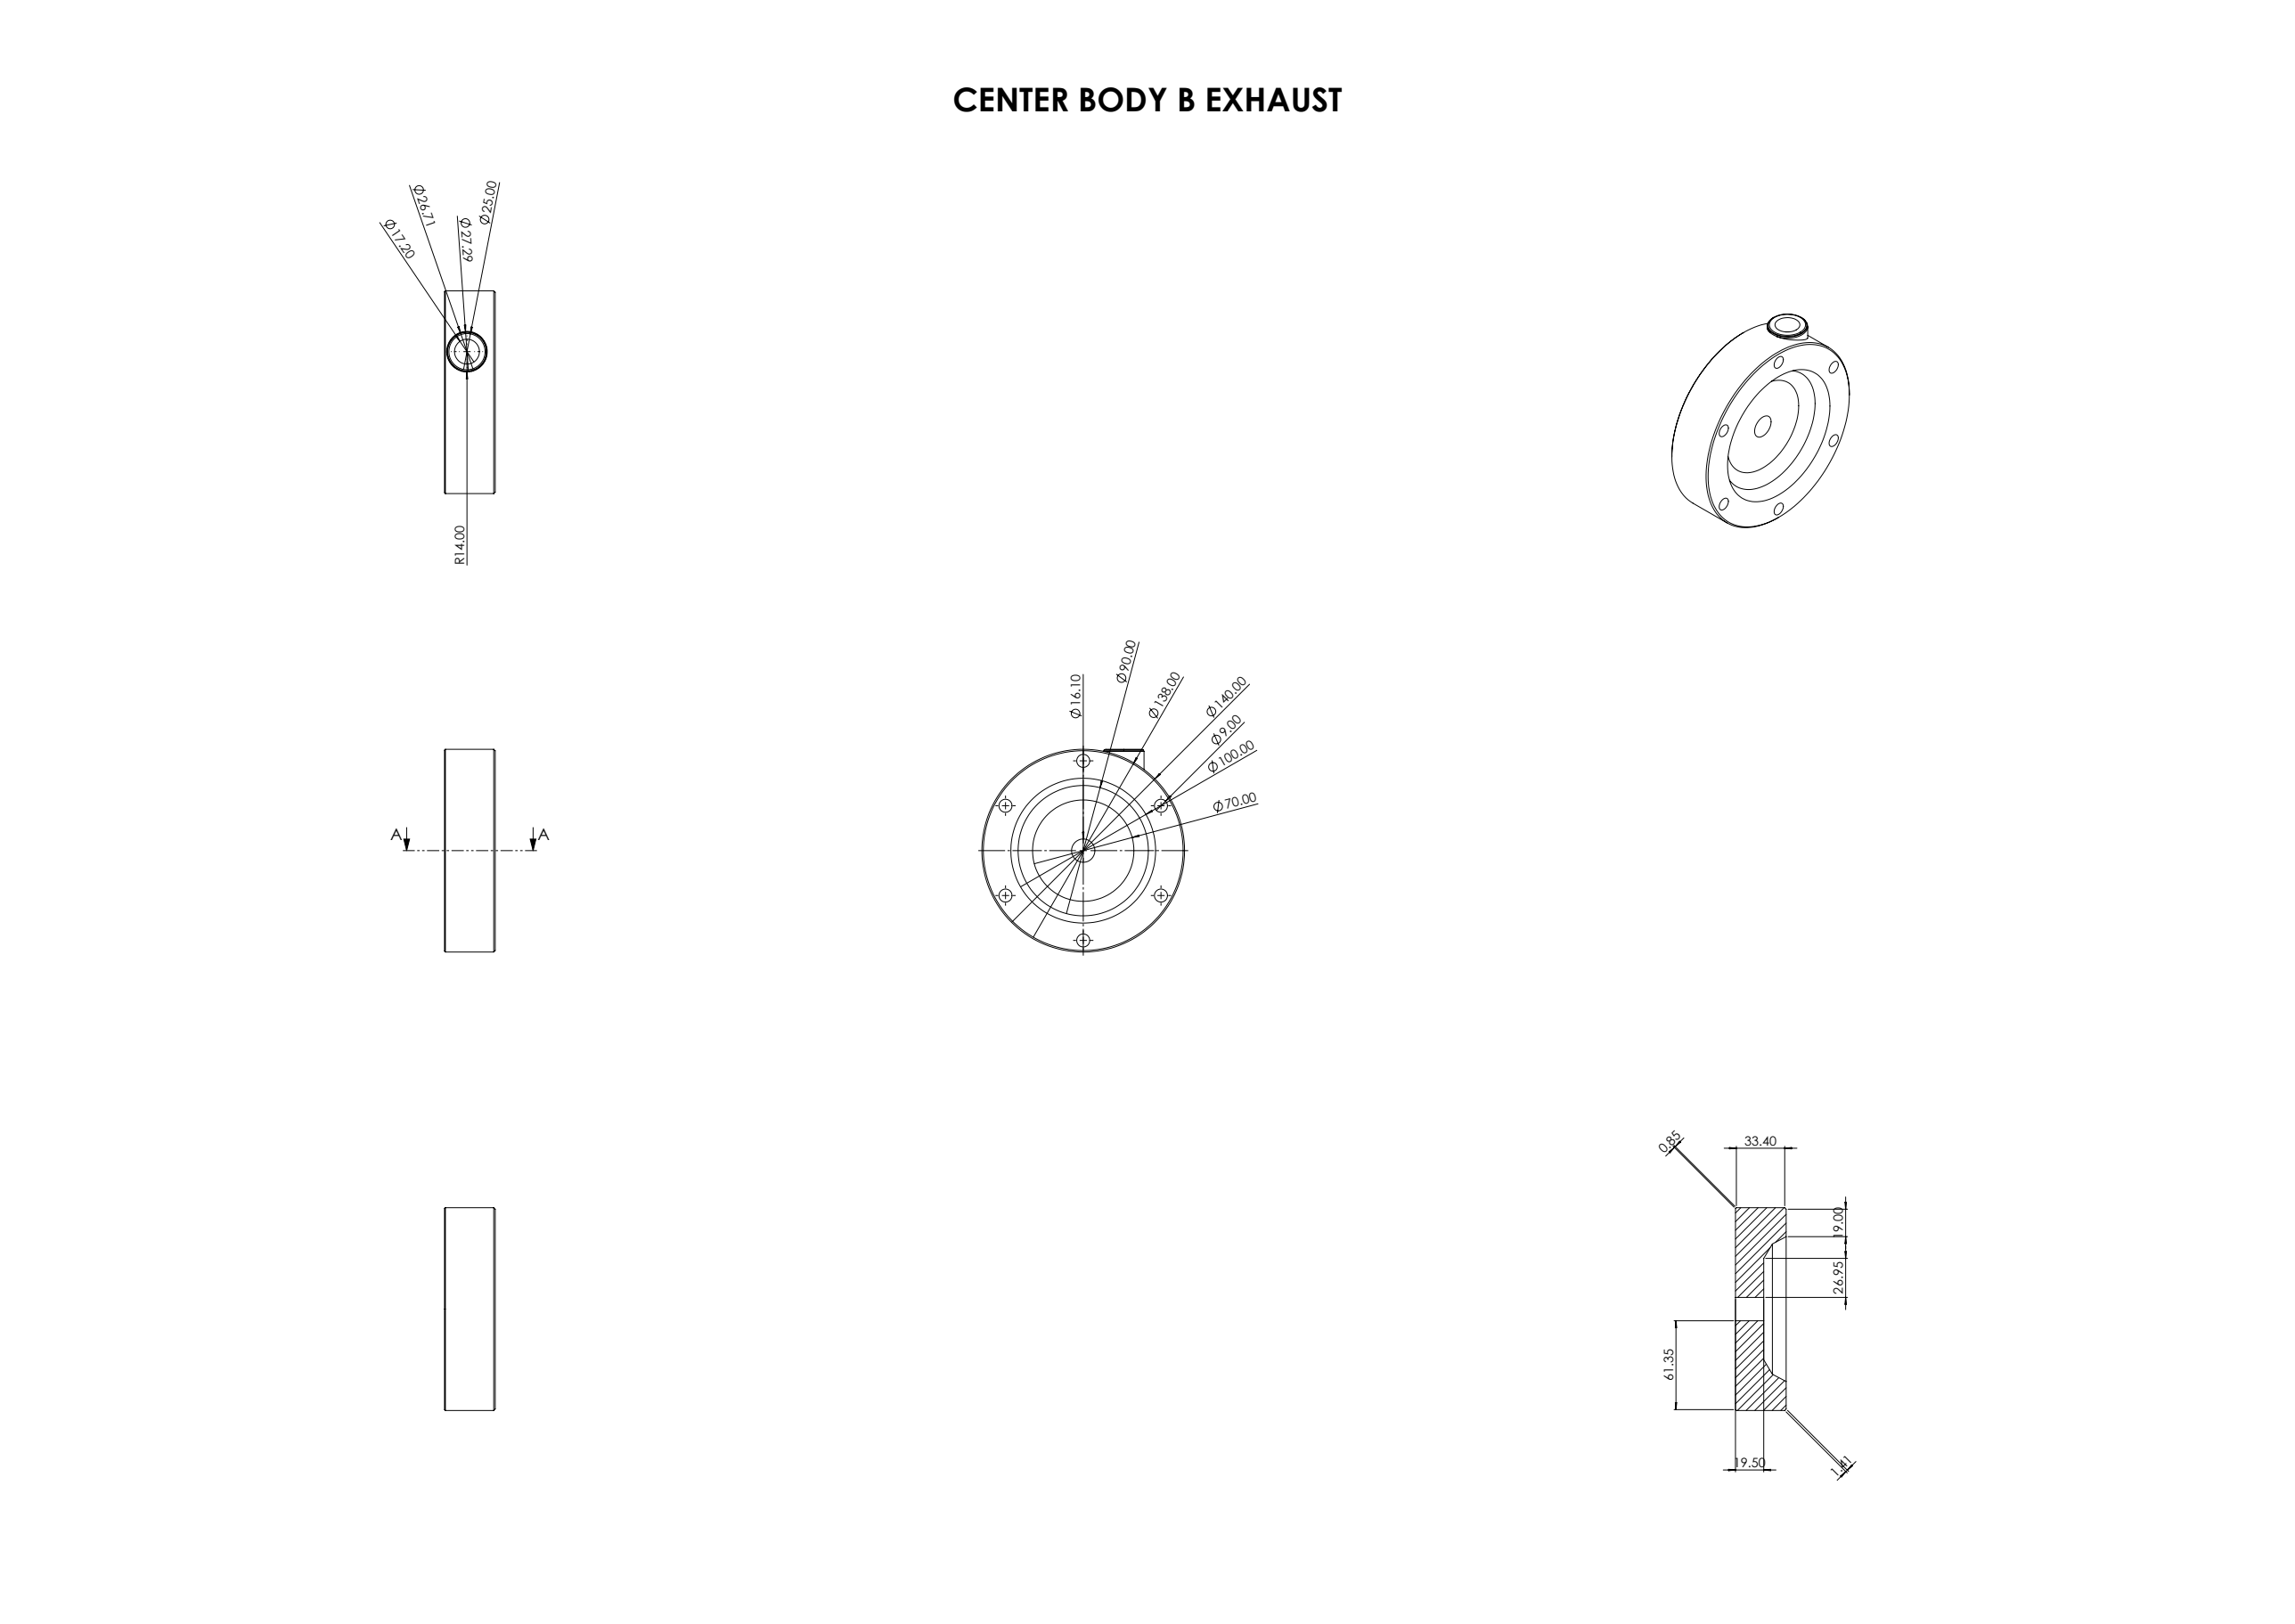
ISO-10303-21;
HEADER;
/* Generated by software containing ST-Developer
 * from STEP Tools, Inc. (www.steptools.com) 
 */

FILE_DESCRIPTION(
/* description */ (''),
/* implementation_level */ '2;1');

FILE_NAME(
/* name */ '03_Center_Body_B_Exhaust.step',
/* time_stamp */ '2026-10-26T06:13:19-07:00',
/* author */ (''),
/* organization */ (''),
/* preprocessor_version */ 'ST-DEVELOPER v20.2',
/* originating_system */ 'Autodesk Translation Framework v15.15.0.0',
/* authorisation */ '');

FILE_SCHEMA (('AUTOMOTIVE_DESIGN { 1 0 10303 214 3 1 1 }','TECHNICAL_DATA_PACKAGING'));
ENDSEC;

DATA;
#10=MECHANICAL_DESIGN_GEOMETRIC_PRESENTATION_REPRESENTATION('',(#299),#56639);
#259=SHAPE_REPRESENTATION_RELATIONSHIP('SRR','None',#56747,#279);
#279=ADVANCED_BREP_SHAPE_REPRESENTATION('',(#319),#56621);
#299=STYLED_ITEM('',(#56894),#319);
#319=MANIFOLD_SOLID_BREP('Body1',#16951);
#459=FACE_BOUND('',#2990,.T.);
#460=FACE_BOUND('',#2994,.T.);
#461=FACE_BOUND('',#2995,.T.);
#462=FACE_BOUND('',#2996,.T.);
#463=FACE_BOUND('',#2997,.T.);
#464=FACE_BOUND('',#2998,.T.);
#465=FACE_BOUND('',#2999,.T.);
#466=FACE_BOUND('',#3000,.T.);
#467=FACE_BOUND('',#3002,.T.);
#468=FACE_BOUND('',#3015,.T.);
#469=FACE_BOUND('',#3016,.T.);
#470=FACE_BOUND('',#3017,.T.);
#471=FACE_BOUND('',#3018,.T.);
#472=FACE_BOUND('',#3019,.T.);
#473=FACE_BOUND('',#3020,.T.);
#474=FACE_BOUND('',#3021,.T.);
#475=FACE_BOUND('',#3025,.T.);
#580=CONICAL_SURFACE('',#17537,12.9267766952966,1.17809724509617);
#581=CONICAL_SURFACE('',#17540,13.5,0.785398163397451);
#582=CONICAL_SURFACE('',#17544,13.8232233047034,0.392699081698724);
#583=CONICAL_SURFACE('',#17547,69.7,0.785398163397444);
#584=CONICAL_SURFACE('',#17579,69.5,0.785398163397448);
#585=CONICAL_SURFACE('',#17583,47.5,0.484477929037023);
#586=CONICAL_SURFACE('',#17585,40.,1.03037682652431);
#843=CIRCLE('',#17538,13.3535533905933);
#844=CIRCLE('',#17539,12.5);
#845=CIRCLE('',#17541,13.6464466094067);
#846=CIRCLE('',#17543,8.6);
#847=CIRCLE('',#17545,14.);
#848=CIRCLE('',#17546,14.);
#849=CIRCLE('',#17548,70.);
#850=CIRCLE('',#17549,70.);
#851=CIRCLE('',#17550,69.4);
#852=CIRCLE('',#17552,4.5);
#853=CIRCLE('',#17553,4.5);
#854=CIRCLE('',#17554,4.5);
#855=CIRCLE('',#17555,4.5);
#856=CIRCLE('',#17556,4.5);
#857=CIRCLE('',#17557,4.5);
#858=CIRCLE('',#17558,8.05);
#859=CIRCLE('',#17560,70.);
#860=CIRCLE('',#17563,8.6);
#861=CIRCLE('',#17566,4.5);
#862=CIRCLE('',#17568,4.5);
#863=CIRCLE('',#17570,4.5);
#864=CIRCLE('',#17572,4.5);
#865=CIRCLE('',#17574,4.5);
#866=CIRCLE('',#17576,4.5);
#867=CIRCLE('',#17578,8.05);
#868=CIRCLE('',#17580,69.);
#869=CIRCLE('',#17582,50.);
#870=CIRCLE('',#17584,45.);
#871=CIRCLE('',#17586,35.);
#1291=CYLINDRICAL_SURFACE('',#17559,70.);
#1292=CYLINDRICAL_SURFACE('',#17561,14.);
#1293=CYLINDRICAL_SURFACE('',#17562,8.6);
#1294=CYLINDRICAL_SURFACE('',#17565,4.5);
#1295=CYLINDRICAL_SURFACE('',#17567,4.5);
#1296=CYLINDRICAL_SURFACE('',#17569,4.5);
#1297=CYLINDRICAL_SURFACE('',#17571,4.5);
#1298=CYLINDRICAL_SURFACE('',#17573,4.5);
#1299=CYLINDRICAL_SURFACE('',#17575,4.5);
#1300=CYLINDRICAL_SURFACE('',#17577,8.05);
#1969=FACE_OUTER_BOUND('',#2987,.T.);
#1970=FACE_OUTER_BOUND('',#2988,.T.);
#1971=FACE_OUTER_BOUND('',#2989,.T.);
#1972=FACE_OUTER_BOUND('',#2991,.T.);
#1973=FACE_OUTER_BOUND('',#2992,.T.);
#1974=FACE_OUTER_BOUND('',#2993,.T.);
#1975=FACE_OUTER_BOUND('',#3001,.T.);
#1976=FACE_OUTER_BOUND('',#3003,.T.);
#1977=FACE_OUTER_BOUND('',#3004,.T.);
#1978=FACE_OUTER_BOUND('',#3005,.T.);
#1979=FACE_OUTER_BOUND('',#3006,.T.);
#1980=FACE_OUTER_BOUND('',#3007,.T.);
#1981=FACE_OUTER_BOUND('',#3008,.T.);
#1982=FACE_OUTER_BOUND('',#3009,.T.);
#1983=FACE_OUTER_BOUND('',#3010,.T.);
#1984=FACE_OUTER_BOUND('',#3011,.T.);
#1985=FACE_OUTER_BOUND('',#3012,.T.);
#1986=FACE_OUTER_BOUND('',#3013,.T.);
#1987=FACE_OUTER_BOUND('',#3014,.T.);
#1988=FACE_OUTER_BOUND('',#3022,.T.);
#1989=FACE_OUTER_BOUND('',#3023,.T.);
#1990=FACE_OUTER_BOUND('',#3024,.T.);
#2987=EDGE_LOOP('',(#11590,#11591,#11592,#11593));
#2988=EDGE_LOOP('',(#11594,#11595,#11596,#11597));
#2989=EDGE_LOOP('',(#11598));
#2990=EDGE_LOOP('',(#11599));
#2991=EDGE_LOOP('',(#11600,#11601,#11602,#11603,#11604,#11605));
#2992=EDGE_LOOP('',(#11606,#11607,#11608,#11609,#11610));
#2993=EDGE_LOOP('',(#11611));
#2994=EDGE_LOOP('',(#11612));
#2995=EDGE_LOOP('',(#11613));
#2996=EDGE_LOOP('',(#11614));
#2997=EDGE_LOOP('',(#11615));
#2998=EDGE_LOOP('',(#11616));
#2999=EDGE_LOOP('',(#11617));
#3000=EDGE_LOOP('',(#11618));
#3001=EDGE_LOOP('',(#11619,#11620,#11621,#11622,#11623));
#3002=EDGE_LOOP('',(#11624,#11625));
#3003=EDGE_LOOP('',(#11626,#11627,#11628));
#3004=EDGE_LOOP('',(#11629,#11630,#11631,#11632));
#3005=EDGE_LOOP('',(#11633));
#3006=EDGE_LOOP('',(#11634,#11635,#11636,#11637));
#3007=EDGE_LOOP('',(#11638,#11639,#11640,#11641));
#3008=EDGE_LOOP('',(#11642,#11643,#11644,#11645));
#3009=EDGE_LOOP('',(#11646,#11647,#11648,#11649));
#3010=EDGE_LOOP('',(#11650,#11651,#11652,#11653));
#3011=EDGE_LOOP('',(#11654,#11655,#11656,#11657));
#3012=EDGE_LOOP('',(#11658,#11659,#11660,#11661));
#3013=EDGE_LOOP('',(#11662,#11663,#11664,#11665));
#3014=EDGE_LOOP('',(#11666));
#3015=EDGE_LOOP('',(#11667));
#3016=EDGE_LOOP('',(#11668));
#3017=EDGE_LOOP('',(#11669));
#3018=EDGE_LOOP('',(#11670));
#3019=EDGE_LOOP('',(#11671));
#3020=EDGE_LOOP('',(#11672));
#3021=EDGE_LOOP('',(#11673));
#3022=EDGE_LOOP('',(#11674,#11675,#11676,#11677));
#3023=EDGE_LOOP('',(#11678,#11679,#11680,#11681));
#3024=EDGE_LOOP('',(#11682));
#3025=EDGE_LOOP('',(#11683));
#4059=LINE('',#24798,#5013);
#4060=LINE('',#24802,#5014);
#4061=LINE('',#24809,#5015);
#4062=LINE('',#24826,#5016);
#4063=LINE('',#24846,#5017);
#4064=LINE('',#24896,#5018);
#4065=LINE('',#24901,#5019);
#4066=LINE('',#24905,#5020);
#4067=LINE('',#24909,#5021);
#4068=LINE('',#24913,#5022);
#4069=LINE('',#24917,#5023);
#4070=LINE('',#24921,#5024);
#4071=LINE('',#24926,#5025);
#4072=LINE('',#24930,#5026);
#4073=LINE('',#24936,#5027);
#4074=LINE('',#24940,#5028);
#5013=VECTOR('',#19645,12.9267766952966);
#5014=VECTOR('',#19650,13.5);
#5015=VECTOR('',#19659,13.8232233047034);
#5016=VECTOR('',#19670,69.7);
#5017=VECTOR('',#19693,70.);
#5018=VECTOR('',#19698,8.6);
#5019=VECTOR('',#19705,4.5);
#5020=VECTOR('',#19710,4.5);
#5021=VECTOR('',#19715,4.5);
#5022=VECTOR('',#19720,4.5);
#5023=VECTOR('',#19725,4.5);
#5024=VECTOR('',#19730,4.5);
#5025=VECTOR('',#19737,8.05);
#5026=VECTOR('',#19742,69.5);
#5027=VECTOR('',#19749,47.5);
#5028=VECTOR('',#19754,40.);
#5879=B_SPLINE_CURVE_WITH_KNOTS('',3,(#24813,#24814,#24815,#24816,#24817,
#24818),.UNSPECIFIED.,.F.,.F.,(4,2,4),(3.40145412174457,3.72577473971897,
4.05009535769338),.UNSPECIFIED.);
#5880=B_SPLINE_CURVE_WITH_KNOTS('',3,(#24847,#24848,#24849,#24850,#24851,
#24852,#24853,#24854,#24855,#24856,#24857,#24858,#24859,#24860,#24861,#24862,
#24863,#24864,#24865,#24866,#24867,#24868,#24869,#24870,#24871,#24872,#24873,
#24874,#24875,#24876,#24877,#24878,#24879,#24880,#24881,#24882,#24883,#24884,
#24885,#24886,#24887,#24888,#24889,#24890,#24891,#24892),.UNSPECIFIED.,
 .F.,.F.,(4,2,2,2,2,2,2,2,2,2,2,2,2,2,2,2,2,2,2,2,2,2,4),(0.330726835810475,
0.524808847269917,1.04961769453983,1.32954893198247,1.6094801694251,1.88941140686773,
2.16934264431036,2.77369676559426,3.37805088687816,3.90945930374807,4.17516351218302,
4.44086772061798,4.70657192905293,4.97227613748788,5.50368455435779,6.10803867564169,
6.71239279692559,6.99232403436822,7.27225527181085,7.55218650925349,7.83211774669612,
8.35692659396604,8.55100860542548),.UNSPECIFIED.);
#6973=VERTEX_POINT('',#24795);
#6974=VERTEX_POINT('',#24797);
#6975=VERTEX_POINT('',#24801);
#6976=VERTEX_POINT('',#24805);
#6977=VERTEX_POINT('',#24808);
#6978=VERTEX_POINT('',#24810);
#6979=VERTEX_POINT('',#24812);
#6980=VERTEX_POINT('',#24821);
#6981=VERTEX_POINT('',#24822);
#6982=VERTEX_POINT('',#24825);
#6983=VERTEX_POINT('',#24829);
#6984=VERTEX_POINT('',#24831);
#6985=VERTEX_POINT('',#24833);
#6986=VERTEX_POINT('',#24835);
#6987=VERTEX_POINT('',#24837);
#6988=VERTEX_POINT('',#24839);
#6989=VERTEX_POINT('',#24841);
#6990=VERTEX_POINT('',#24844);
#6991=VERTEX_POINT('',#24895);
#6992=VERTEX_POINT('',#24900);
#6993=VERTEX_POINT('',#24904);
#6994=VERTEX_POINT('',#24908);
#6995=VERTEX_POINT('',#24912);
#6996=VERTEX_POINT('',#24916);
#6997=VERTEX_POINT('',#24920);
#6998=VERTEX_POINT('',#24924);
#6999=VERTEX_POINT('',#24928);
#7000=VERTEX_POINT('',#24932);
#7001=VERTEX_POINT('',#24935);
#7002=VERTEX_POINT('',#24939);
#8702=EDGE_CURVE('',#6973,#6973,#843,.T.);
#8703=EDGE_CURVE('',#6973,#6974,#4059,.T.);
#8704=EDGE_CURVE('',#6974,#6974,#844,.T.);
#8705=EDGE_CURVE('',#6973,#6975,#4060,.T.);
#8706=EDGE_CURVE('',#6975,#6975,#845,.T.);
#8707=EDGE_CURVE('',#6976,#6976,#846,.T.);
#8708=EDGE_CURVE('',#6975,#6977,#4061,.T.);
#8709=EDGE_CURVE('',#6977,#6978,#847,.T.);
#8710=EDGE_CURVE('',#6979,#6978,#5879,.T.);
#8711=EDGE_CURVE('',#6979,#6977,#848,.T.);
#8712=EDGE_CURVE('',#6980,#6981,#849,.T.);
#8713=EDGE_CURVE('',#6981,#6980,#850,.T.);
#8714=EDGE_CURVE('',#6980,#6982,#4062,.T.);
#8715=EDGE_CURVE('',#6982,#6982,#851,.T.);
#8716=EDGE_CURVE('',#6983,#6983,#852,.T.);
#8717=EDGE_CURVE('',#6984,#6984,#853,.T.);
#8718=EDGE_CURVE('',#6985,#6985,#854,.T.);
#8719=EDGE_CURVE('',#6986,#6986,#855,.T.);
#8720=EDGE_CURVE('',#6987,#6987,#856,.T.);
#8721=EDGE_CURVE('',#6988,#6988,#857,.T.);
#8722=EDGE_CURVE('',#6989,#6989,#858,.T.);
#8723=EDGE_CURVE('',#6990,#6990,#859,.T.);
#8724=EDGE_CURVE('',#6990,#6981,#4063,.T.);
#8725=EDGE_CURVE('',#6978,#6979,#5880,.T.);
#8726=EDGE_CURVE('',#6976,#6991,#4064,.T.);
#8727=EDGE_CURVE('',#6991,#6991,#860,.T.);
#8728=EDGE_CURVE('',#6983,#6992,#4065,.T.);
#8729=EDGE_CURVE('',#6992,#6992,#861,.T.);
#8730=EDGE_CURVE('',#6984,#6993,#4066,.T.);
#8731=EDGE_CURVE('',#6993,#6993,#862,.T.);
#8732=EDGE_CURVE('',#6985,#6994,#4067,.T.);
#8733=EDGE_CURVE('',#6994,#6994,#863,.T.);
#8734=EDGE_CURVE('',#6986,#6995,#4068,.T.);
#8735=EDGE_CURVE('',#6995,#6995,#864,.T.);
#8736=EDGE_CURVE('',#6987,#6996,#4069,.T.);
#8737=EDGE_CURVE('',#6996,#6996,#865,.T.);
#8738=EDGE_CURVE('',#6988,#6997,#4070,.T.);
#8739=EDGE_CURVE('',#6997,#6997,#866,.T.);
#8740=EDGE_CURVE('',#6998,#6998,#867,.T.);
#8741=EDGE_CURVE('',#6998,#6989,#4071,.T.);
#8742=EDGE_CURVE('',#6999,#6999,#868,.T.);
#8743=EDGE_CURVE('',#6999,#6990,#4072,.T.);
#8744=EDGE_CURVE('',#7000,#7000,#869,.T.);
#8745=EDGE_CURVE('',#7000,#7001,#4073,.T.);
#8746=EDGE_CURVE('',#7001,#7001,#870,.T.);
#8747=EDGE_CURVE('',#7001,#7002,#4074,.T.);
#8748=EDGE_CURVE('',#7002,#7002,#871,.T.);
#11590=ORIENTED_EDGE('',*,*,#8702,.T.);
#11591=ORIENTED_EDGE('',*,*,#8703,.T.);
#11592=ORIENTED_EDGE('',*,*,#8704,.T.);
#11593=ORIENTED_EDGE('',*,*,#8703,.F.);
#11594=ORIENTED_EDGE('',*,*,#8702,.F.);
#11595=ORIENTED_EDGE('',*,*,#8705,.T.);
#11596=ORIENTED_EDGE('',*,*,#8706,.F.);
#11597=ORIENTED_EDGE('',*,*,#8705,.F.);
#11598=ORIENTED_EDGE('',*,*,#8704,.F.);
#11599=ORIENTED_EDGE('',*,*,#8707,.T.);
#11600=ORIENTED_EDGE('',*,*,#8706,.T.);
#11601=ORIENTED_EDGE('',*,*,#8708,.T.);
#11602=ORIENTED_EDGE('',*,*,#8709,.T.);
#11603=ORIENTED_EDGE('',*,*,#8710,.F.);
#11604=ORIENTED_EDGE('',*,*,#8711,.T.);
#11605=ORIENTED_EDGE('',*,*,#8708,.F.);
#11606=ORIENTED_EDGE('',*,*,#8712,.T.);
#11607=ORIENTED_EDGE('',*,*,#8713,.T.);
#11608=ORIENTED_EDGE('',*,*,#8714,.T.);
#11609=ORIENTED_EDGE('',*,*,#8715,.T.);
#11610=ORIENTED_EDGE('',*,*,#8714,.F.);
#11611=ORIENTED_EDGE('',*,*,#8715,.F.);
#11612=ORIENTED_EDGE('',*,*,#8716,.T.);
#11613=ORIENTED_EDGE('',*,*,#8717,.T.);
#11614=ORIENTED_EDGE('',*,*,#8718,.T.);
#11615=ORIENTED_EDGE('',*,*,#8719,.T.);
#11616=ORIENTED_EDGE('',*,*,#8720,.T.);
#11617=ORIENTED_EDGE('',*,*,#8721,.T.);
#11618=ORIENTED_EDGE('',*,*,#8722,.T.);
#11619=ORIENTED_EDGE('',*,*,#8723,.F.);
#11620=ORIENTED_EDGE('',*,*,#8724,.T.);
#11621=ORIENTED_EDGE('',*,*,#8712,.F.);
#11622=ORIENTED_EDGE('',*,*,#8713,.F.);
#11623=ORIENTED_EDGE('',*,*,#8724,.F.);
#11624=ORIENTED_EDGE('',*,*,#8725,.T.);
#11625=ORIENTED_EDGE('',*,*,#8710,.T.);
#11626=ORIENTED_EDGE('',*,*,#8711,.F.);
#11627=ORIENTED_EDGE('',*,*,#8725,.F.);
#11628=ORIENTED_EDGE('',*,*,#8709,.F.);
#11629=ORIENTED_EDGE('',*,*,#8707,.F.);
#11630=ORIENTED_EDGE('',*,*,#8726,.T.);
#11631=ORIENTED_EDGE('',*,*,#8727,.T.);
#11632=ORIENTED_EDGE('',*,*,#8726,.F.);
#11633=ORIENTED_EDGE('',*,*,#8727,.F.);
#11634=ORIENTED_EDGE('',*,*,#8716,.F.);
#11635=ORIENTED_EDGE('',*,*,#8728,.T.);
#11636=ORIENTED_EDGE('',*,*,#8729,.F.);
#11637=ORIENTED_EDGE('',*,*,#8728,.F.);
#11638=ORIENTED_EDGE('',*,*,#8717,.F.);
#11639=ORIENTED_EDGE('',*,*,#8730,.T.);
#11640=ORIENTED_EDGE('',*,*,#8731,.F.);
#11641=ORIENTED_EDGE('',*,*,#8730,.F.);
#11642=ORIENTED_EDGE('',*,*,#8718,.F.);
#11643=ORIENTED_EDGE('',*,*,#8732,.T.);
#11644=ORIENTED_EDGE('',*,*,#8733,.F.);
#11645=ORIENTED_EDGE('',*,*,#8732,.F.);
#11646=ORIENTED_EDGE('',*,*,#8719,.F.);
#11647=ORIENTED_EDGE('',*,*,#8734,.T.);
#11648=ORIENTED_EDGE('',*,*,#8735,.F.);
#11649=ORIENTED_EDGE('',*,*,#8734,.F.);
#11650=ORIENTED_EDGE('',*,*,#8720,.F.);
#11651=ORIENTED_EDGE('',*,*,#8736,.T.);
#11652=ORIENTED_EDGE('',*,*,#8737,.F.);
#11653=ORIENTED_EDGE('',*,*,#8736,.F.);
#11654=ORIENTED_EDGE('',*,*,#8721,.F.);
#11655=ORIENTED_EDGE('',*,*,#8738,.T.);
#11656=ORIENTED_EDGE('',*,*,#8739,.F.);
#11657=ORIENTED_EDGE('',*,*,#8738,.F.);
#11658=ORIENTED_EDGE('',*,*,#8740,.T.);
#11659=ORIENTED_EDGE('',*,*,#8741,.T.);
#11660=ORIENTED_EDGE('',*,*,#8722,.F.);
#11661=ORIENTED_EDGE('',*,*,#8741,.F.);
#11662=ORIENTED_EDGE('',*,*,#8742,.F.);
#11663=ORIENTED_EDGE('',*,*,#8743,.T.);
#11664=ORIENTED_EDGE('',*,*,#8723,.T.);
#11665=ORIENTED_EDGE('',*,*,#8743,.F.);
#11666=ORIENTED_EDGE('',*,*,#8742,.T.);
#11667=ORIENTED_EDGE('',*,*,#8744,.F.);
#11668=ORIENTED_EDGE('',*,*,#8739,.T.);
#11669=ORIENTED_EDGE('',*,*,#8737,.T.);
#11670=ORIENTED_EDGE('',*,*,#8735,.T.);
#11671=ORIENTED_EDGE('',*,*,#8733,.T.);
#11672=ORIENTED_EDGE('',*,*,#8731,.T.);
#11673=ORIENTED_EDGE('',*,*,#8729,.T.);
#11674=ORIENTED_EDGE('',*,*,#8744,.T.);
#11675=ORIENTED_EDGE('',*,*,#8745,.T.);
#11676=ORIENTED_EDGE('',*,*,#8746,.F.);
#11677=ORIENTED_EDGE('',*,*,#8745,.F.);
#11678=ORIENTED_EDGE('',*,*,#8746,.T.);
#11679=ORIENTED_EDGE('',*,*,#8747,.T.);
#11680=ORIENTED_EDGE('',*,*,#8748,.F.);
#11681=ORIENTED_EDGE('',*,*,#8747,.F.);
#11682=ORIENTED_EDGE('',*,*,#8748,.T.);
#11683=ORIENTED_EDGE('',*,*,#8740,.F.);
#15768=PLANE('',#17542);
#15769=PLANE('',#17551);
#15770=PLANE('',#17564);
#15771=PLANE('',#17581);
#15772=PLANE('',#17587);
#16140=ADVANCED_FACE('',(#1969),#580,.T.);
#16141=ADVANCED_FACE('',(#1970),#581,.T.);
#16142=ADVANCED_FACE('',(#1971,#459),#15768,.T.);
#16143=ADVANCED_FACE('',(#1972),#582,.T.);
#16144=ADVANCED_FACE('',(#1973),#583,.T.);
#16145=ADVANCED_FACE('',(#1974,#460,#461,#462,#463,#464,#465,#466),#15769,
 .T.);
#16146=ADVANCED_FACE('',(#1975,#467),#1291,.T.);
#16147=ADVANCED_FACE('',(#1976),#1292,.T.);
#16148=ADVANCED_FACE('',(#1977),#1293,.F.);
#16149=ADVANCED_FACE('',(#1978),#15770,.T.);
#16150=ADVANCED_FACE('',(#1979),#1294,.F.);
#16151=ADVANCED_FACE('',(#1980),#1295,.F.);
#16152=ADVANCED_FACE('',(#1981),#1296,.F.);
#16153=ADVANCED_FACE('',(#1982),#1297,.F.);
#16154=ADVANCED_FACE('',(#1983),#1298,.F.);
#16155=ADVANCED_FACE('',(#1984),#1299,.F.);
#16156=ADVANCED_FACE('',(#1985),#1300,.F.);
#16157=ADVANCED_FACE('',(#1986),#584,.T.);
#16158=ADVANCED_FACE('',(#1987,#468,#469,#470,#471,#472,#473,#474),#15771,
 .T.);
#16159=ADVANCED_FACE('',(#1988),#585,.F.);
#16160=ADVANCED_FACE('',(#1989),#586,.F.);
#16161=ADVANCED_FACE('',(#1990,#475),#15772,.T.);
#16951=CLOSED_SHELL('',(#16140,#16141,#16142,#16143,#16144,#16145,#16146,
#16147,#16148,#16149,#16150,#16151,#16152,#16153,#16154,#16155,#16156,#16157,
#16158,#16159,#16160,#16161));
#17536=AXIS2_PLACEMENT_3D('',#24793,#19639,#19640);
#17537=AXIS2_PLACEMENT_3D('',#24794,#19641,#19642);
#17538=AXIS2_PLACEMENT_3D('',#24796,#19643,#19644);
#17539=AXIS2_PLACEMENT_3D('',#24799,#19646,#19647);
#17540=AXIS2_PLACEMENT_3D('',#24800,#19648,#19649);
#17541=AXIS2_PLACEMENT_3D('',#24803,#19651,#19652);
#17542=AXIS2_PLACEMENT_3D('',#24804,#19653,#19654);
#17543=AXIS2_PLACEMENT_3D('',#24806,#19655,#19656);
#17544=AXIS2_PLACEMENT_3D('',#24807,#19657,#19658);
#17545=AXIS2_PLACEMENT_3D('',#24811,#19660,#19661);
#17546=AXIS2_PLACEMENT_3D('',#24819,#19662,#19663);
#17547=AXIS2_PLACEMENT_3D('',#24820,#19664,#19665);
#17548=AXIS2_PLACEMENT_3D('',#24823,#19666,#19667);
#17549=AXIS2_PLACEMENT_3D('',#24824,#19668,#19669);
#17550=AXIS2_PLACEMENT_3D('',#24827,#19671,#19672);
#17551=AXIS2_PLACEMENT_3D('',#24828,#19673,#19674);
#17552=AXIS2_PLACEMENT_3D('',#24830,#19675,#19676);
#17553=AXIS2_PLACEMENT_3D('',#24832,#19677,#19678);
#17554=AXIS2_PLACEMENT_3D('',#24834,#19679,#19680);
#17555=AXIS2_PLACEMENT_3D('',#24836,#19681,#19682);
#17556=AXIS2_PLACEMENT_3D('',#24838,#19683,#19684);
#17557=AXIS2_PLACEMENT_3D('',#24840,#19685,#19686);
#17558=AXIS2_PLACEMENT_3D('',#24842,#19687,#19688);
#17559=AXIS2_PLACEMENT_3D('',#24843,#19689,#19690);
#17560=AXIS2_PLACEMENT_3D('',#24845,#19691,#19692);
#17561=AXIS2_PLACEMENT_3D('',#24893,#19694,#19695);
#17562=AXIS2_PLACEMENT_3D('',#24894,#19696,#19697);
#17563=AXIS2_PLACEMENT_3D('',#24897,#19699,#19700);
#17564=AXIS2_PLACEMENT_3D('',#24898,#19701,#19702);
#17565=AXIS2_PLACEMENT_3D('',#24899,#19703,#19704);
#17566=AXIS2_PLACEMENT_3D('',#24902,#19706,#19707);
#17567=AXIS2_PLACEMENT_3D('',#24903,#19708,#19709);
#17568=AXIS2_PLACEMENT_3D('',#24906,#19711,#19712);
#17569=AXIS2_PLACEMENT_3D('',#24907,#19713,#19714);
#17570=AXIS2_PLACEMENT_3D('',#24910,#19716,#19717);
#17571=AXIS2_PLACEMENT_3D('',#24911,#19718,#19719);
#17572=AXIS2_PLACEMENT_3D('',#24914,#19721,#19722);
#17573=AXIS2_PLACEMENT_3D('',#24915,#19723,#19724);
#17574=AXIS2_PLACEMENT_3D('',#24918,#19726,#19727);
#17575=AXIS2_PLACEMENT_3D('',#24919,#19728,#19729);
#17576=AXIS2_PLACEMENT_3D('',#24922,#19731,#19732);
#17577=AXIS2_PLACEMENT_3D('',#24923,#19733,#19734);
#17578=AXIS2_PLACEMENT_3D('',#24925,#19735,#19736);
#17579=AXIS2_PLACEMENT_3D('',#24927,#19738,#19739);
#17580=AXIS2_PLACEMENT_3D('',#24929,#19740,#19741);
#17581=AXIS2_PLACEMENT_3D('',#24931,#19743,#19744);
#17582=AXIS2_PLACEMENT_3D('',#24933,#19745,#19746);
#17583=AXIS2_PLACEMENT_3D('',#24934,#19747,#19748);
#17584=AXIS2_PLACEMENT_3D('',#24937,#19750,#19751);
#17585=AXIS2_PLACEMENT_3D('',#24938,#19752,#19753);
#17586=AXIS2_PLACEMENT_3D('',#24941,#19755,#19756);
#17587=AXIS2_PLACEMENT_3D('',#24942,#19757,#19758);
#19639=DIRECTION('axis',(0.,0.,1.));
#19640=DIRECTION('refdir',(1.,0.,0.));
#19641=DIRECTION('center_axis',(0.,-1.,0.));
#19642=DIRECTION('ref_axis',(1.,3.43542106681276E-16,0.));
#19643=DIRECTION('center_axis',(-6.65125149629304E-16,1.,0.));
#19644=DIRECTION('ref_axis',(1.,6.65125149629305E-16,0.));
#19645=DIRECTION('',(0.923879532511289,0.382683432365085,1.1314261122877E-16));
#19646=DIRECTION('center_axis',(0.,-1.,0.));
#19647=DIRECTION('ref_axis',(1.,0.,0.));
#19648=DIRECTION('center_axis',(0.,-1.,0.));
#19649=DIRECTION('ref_axis',(1.,0.,0.));
#19650=DIRECTION('',(-0.707106781186549,-0.707106781186546,8.65956056235495E-17));
#19651=DIRECTION('center_axis',(0.,-1.,0.));
#19652=DIRECTION('ref_axis',(1.,0.,0.));
#19653=DIRECTION('center_axis',(0.,1.,0.));
#19654=DIRECTION('ref_axis',(1.,0.,0.));
#19655=DIRECTION('center_axis',(0.,-1.,0.));
#19656=DIRECTION('ref_axis',(1.,0.,0.));
#19657=DIRECTION('center_axis',(0.,-1.,0.));
#19658=DIRECTION('ref_axis',(1.,0.,0.));
#19659=DIRECTION('',(-0.38268343236509,-0.923879532511287,4.6865204053263E-17));
#19660=DIRECTION('center_axis',(0.,1.,0.));
#19661=DIRECTION('ref_axis',(1.,0.,0.));
#19662=DIRECTION('center_axis',(0.,1.,0.));
#19663=DIRECTION('ref_axis',(1.,0.,0.));
#19664=DIRECTION('center_axis',(1.,0.,0.));
#19665=DIRECTION('ref_axis',(0.,-1.,0.));
#19666=DIRECTION('center_axis',(-1.,0.,0.));
#19667=DIRECTION('ref_axis',(0.,-1.,0.));
#19668=DIRECTION('center_axis',(-1.,0.,0.));
#19669=DIRECTION('ref_axis',(0.,-1.,0.));
#19670=DIRECTION('',(-0.70710678118655,-0.707106781186545,-8.6595605623549E-17));
#19671=DIRECTION('center_axis',(1.,0.,0.));
#19672=DIRECTION('ref_axis',(0.,-1.,0.));
#19673=DIRECTION('center_axis',(-1.,0.,0.));
#19674=DIRECTION('ref_axis',(0.,0.,1.));
#19675=DIRECTION('center_axis',(1.,0.,0.));
#19676=DIRECTION('ref_axis',(0.,0.,-1.));
#19677=DIRECTION('center_axis',(1.,0.,0.));
#19678=DIRECTION('ref_axis',(0.,0.,-1.));
#19679=DIRECTION('center_axis',(1.,0.,0.));
#19680=DIRECTION('ref_axis',(0.,0.,-1.));
#19681=DIRECTION('center_axis',(1.,0.,0.));
#19682=DIRECTION('ref_axis',(0.,0.,-1.));
#19683=DIRECTION('center_axis',(1.,0.,0.));
#19684=DIRECTION('ref_axis',(0.,0.,-1.));
#19685=DIRECTION('center_axis',(1.,0.,0.));
#19686=DIRECTION('ref_axis',(0.,0.,-1.));
#19687=DIRECTION('center_axis',(1.,0.,0.));
#19688=DIRECTION('ref_axis',(0.,0.,-1.));
#19689=DIRECTION('center_axis',(1.,0.,0.));
#19690=DIRECTION('ref_axis',(0.,1.,0.));
#19691=DIRECTION('center_axis',(1.,0.,0.));
#19692=DIRECTION('ref_axis',(0.,0.,-1.));
#19693=DIRECTION('',(-1.,0.,0.));
#19694=DIRECTION('center_axis',(0.,1.,0.));
#19695=DIRECTION('ref_axis',(9.49410759657493E-16,0.,-1.));
#19696=DIRECTION('center_axis',(0.,-1.,0.));
#19697=DIRECTION('ref_axis',(1.,0.,0.));
#19698=DIRECTION('',(0.,-1.,0.));
#19699=DIRECTION('center_axis',(0.,-1.,0.));
#19700=DIRECTION('ref_axis',(1.,0.,0.));
#19701=DIRECTION('center_axis',(0.,1.,0.));
#19702=DIRECTION('ref_axis',(1.,0.,0.));
#19703=DIRECTION('center_axis',(1.,0.,0.));
#19704=DIRECTION('ref_axis',(0.,0.,-1.));
#19705=DIRECTION('',(1.,0.,0.));
#19706=DIRECTION('center_axis',(-1.,0.,0.));
#19707=DIRECTION('ref_axis',(0.,0.,-1.));
#19708=DIRECTION('center_axis',(1.,0.,0.));
#19709=DIRECTION('ref_axis',(0.,0.,-1.));
#19710=DIRECTION('',(1.,0.,0.));
#19711=DIRECTION('center_axis',(-1.,0.,0.));
#19712=DIRECTION('ref_axis',(0.,0.,-1.));
#19713=DIRECTION('center_axis',(1.,0.,0.));
#19714=DIRECTION('ref_axis',(0.,0.,-1.));
#19715=DIRECTION('',(1.,0.,0.));
#19716=DIRECTION('center_axis',(-1.,0.,0.));
#19717=DIRECTION('ref_axis',(0.,0.,-1.));
#19718=DIRECTION('center_axis',(1.,0.,0.));
#19719=DIRECTION('ref_axis',(0.,0.,-1.));
#19720=DIRECTION('',(1.,0.,0.));
#19721=DIRECTION('center_axis',(-1.,0.,0.));
#19722=DIRECTION('ref_axis',(0.,0.,-1.));
#19723=DIRECTION('center_axis',(1.,0.,0.));
#19724=DIRECTION('ref_axis',(0.,0.,-1.));
#19725=DIRECTION('',(1.,0.,0.));
#19726=DIRECTION('center_axis',(-1.,0.,0.));
#19727=DIRECTION('ref_axis',(0.,0.,-1.));
#19728=DIRECTION('center_axis',(1.,0.,0.));
#19729=DIRECTION('ref_axis',(0.,0.,-1.));
#19730=DIRECTION('',(1.,0.,0.));
#19731=DIRECTION('center_axis',(-1.,0.,0.));
#19732=DIRECTION('ref_axis',(0.,0.,-1.));
#19733=DIRECTION('center_axis',(1.,0.,0.));
#19734=DIRECTION('ref_axis',(0.,1.,0.));
#19735=DIRECTION('center_axis',(1.,0.,0.));
#19736=DIRECTION('ref_axis',(0.,0.,-1.));
#19737=DIRECTION('',(-1.,0.,0.));
#19738=DIRECTION('center_axis',(-1.,0.,0.));
#19739=DIRECTION('ref_axis',(0.,1.,0.));
#19740=DIRECTION('center_axis',(1.,0.,0.));
#19741=DIRECTION('ref_axis',(0.,0.,-1.));
#19742=DIRECTION('',(-0.707106781186547,-0.707106781186547,-8.65956056235493E-17));
#19743=DIRECTION('center_axis',(1.,0.,0.));
#19744=DIRECTION('ref_axis',(0.,0.,-1.));
#19745=DIRECTION('center_axis',(1.,0.,0.));
#19746=DIRECTION('ref_axis',(0.,0.,-1.));
#19747=DIRECTION('center_axis',(1.,0.,0.));
#19748=DIRECTION('ref_axis',(0.,1.,0.));
#19749=DIRECTION('',(-0.884918222381982,0.465746432832622,5.70374878182769E-17));
#19750=DIRECTION('center_axis',(1.,0.,0.));
#19751=DIRECTION('ref_axis',(0.,0.,-1.));
#19752=DIRECTION('center_axis',(1.,0.,0.));
#19753=DIRECTION('ref_axis',(0.,1.,0.));
#19754=DIRECTION('',(-0.514495755427527,0.857492925712544,1.05012596676537E-16));
#19755=DIRECTION('center_axis',(1.,0.,0.));
#19756=DIRECTION('ref_axis',(0.,0.,-1.));
#19757=DIRECTION('center_axis',(1.,0.,0.));
#19758=DIRECTION('ref_axis',(0.,0.,-1.));
#24793=CARTESIAN_POINT('',(0.,0.,0.));
#24794=CARTESIAN_POINT('Origin',(16.,69.8232233047034,-28.));
#24795=CARTESIAN_POINT('',(2.64644660940673,69.6464466094067,-28.));
#24796=CARTESIAN_POINT('Origin',(16.,69.6464466094067,-28.));
#24797=CARTESIAN_POINT('',(3.5,70.,-28.));
#24798=CARTESIAN_POINT('',(3.07322330470337,69.8232233047034,-28.));
#24799=CARTESIAN_POINT('Origin',(16.,70.,-28.));
#24800=CARTESIAN_POINT('Origin',(16.,69.5,-28.));
#24801=CARTESIAN_POINT('',(2.35355339059327,69.3535533905933,-28.));
#24802=CARTESIAN_POINT('',(2.5,69.5,-28.));
#24803=CARTESIAN_POINT('Origin',(16.,69.3535533905933,-28.));
#24804=CARTESIAN_POINT('Origin',(16.,70.,-28.));
#24805=CARTESIAN_POINT('',(7.4,70.,-28.));
#24806=CARTESIAN_POINT('Origin',(16.,70.,-28.));
#24807=CARTESIAN_POINT('Origin',(16.,68.9267766952966,-28.));
#24808=CARTESIAN_POINT('',(1.99999999999998,68.5,-28.));
#24809=CARTESIAN_POINT('',(2.17677669529664,68.9267766952966,-28.));
#24810=CARTESIAN_POINT('',(12.6224302964435,68.5,-14.4135353053998));
#24811=CARTESIAN_POINT('Origin',(16.,68.5,-28.));
#24812=CARTESIAN_POINT('',(19.3775697035565,68.5,-14.4135353053998));
#24813=CARTESIAN_POINT('Ctrl Pts',(19.3775697035564,68.5,-14.4135353053998));
#24814=CARTESIAN_POINT('Ctrl Pts',(18.2401900876009,68.5545924215965,-14.1540860585547));
#24815=CARTESIAN_POINT('Ctrl Pts',(17.0810687265813,68.5790231734206,-14.0327324701726));
#24816=CARTESIAN_POINT('Ctrl Pts',(14.9189312734187,68.5790231734206,-14.0327324701726));
#24817=CARTESIAN_POINT('Ctrl Pts',(13.7598099123991,68.5545924215965,-14.1540860585547));
#24818=CARTESIAN_POINT('Ctrl Pts',(12.6224302964436,68.5,-14.4135353053998));
#24819=CARTESIAN_POINT('Origin',(16.,68.5,-28.));
#24820=CARTESIAN_POINT('Origin',(0.8,0.,0.));
#24821=CARTESIAN_POINT('',(1.1,70.,-8.57252759403147E-15));
#24822=CARTESIAN_POINT('',(1.1,-70.,-8.57252759403147E-15));
#24823=CARTESIAN_POINT('Origin',(1.1,0.,0.));
#24824=CARTESIAN_POINT('Origin',(1.1,0.,0.));
#24825=CARTESIAN_POINT('',(0.5,69.4,8.49904878608263E-15));
#24826=CARTESIAN_POINT('',(0.8,69.7,8.53578819005705E-15));
#24827=CARTESIAN_POINT('Origin',(0.5,0.,0.));
#24828=CARTESIAN_POINT('Origin',(0.5,70.,0.));
#24829=CARTESIAN_POINT('',(0.5,-31.,-49.1935750346352));
#24830=CARTESIAN_POINT('Origin',(0.5,-31.,-53.6935750346352));
#24831=CARTESIAN_POINT('',(0.5,62.,4.5));
#24832=CARTESIAN_POINT('Origin',(0.5,62.,0.));
#24833=CARTESIAN_POINT('',(0.5,31.,58.1935750346352));
#24834=CARTESIAN_POINT('Origin',(0.5,31.,53.6935750346352));
#24835=CARTESIAN_POINT('',(0.5,-31.,58.1935750346352));
#24836=CARTESIAN_POINT('Origin',(0.5,-31.,53.6935750346352));
#24837=CARTESIAN_POINT('',(0.5,-62.,4.50000000000001));
#24838=CARTESIAN_POINT('Origin',(0.5,-62.,7.59281015471359E-15));
#24839=CARTESIAN_POINT('',(0.5,31.,-49.1935750346352));
#24840=CARTESIAN_POINT('Origin',(0.5,31.,-53.6935750346352));
#24841=CARTESIAN_POINT('',(0.5,-8.05,-9.85840673313619E-16));
#24842=CARTESIAN_POINT('Origin',(0.5,0.,0.));
#24843=CARTESIAN_POINT('Origin',(17.5,0.,0.));
#24844=CARTESIAN_POINT('',(34.5,-70.,-8.57252759403147E-15));
#24845=CARTESIAN_POINT('Origin',(34.5,0.,0.));
#24846=CARTESIAN_POINT('',(17.5,-70.,-8.57252759403147E-15));
#24847=CARTESIAN_POINT('Ctrl Pts',(12.6224302964435,68.5,-14.4135353053998));
#24848=CARTESIAN_POINT('Ctrl Pts',(11.961651315758,68.4654352022338,-14.5778037237174));
#24849=CARTESIAN_POINT('Ctrl Pts',(11.3086498622677,68.4198540566006,-14.7917039729986));
#24850=CARTESIAN_POINT('Ctrl Pts',(8.96544243852918,68.2077217953467,-15.7551700622329));
#24851=CARTESIAN_POINT('Ctrl Pts',(7.4085187040214,67.9622849181329,-16.8132432389867));
#24852=CARTESIAN_POINT('Ctrl Pts',(5.52865282034834,67.4697026576732,-18.662322985451));
#24853=CARTESIAN_POINT('Ctrl Pts',(4.92185391533271,67.2665458430878,-19.3877268629585));
#24854=CARTESIAN_POINT('Ctrl Pts',(3.86308556320828,66.7940167052205,-20.9578499606675));
#24855=CARTESIAN_POINT('Ctrl Pts',(3.41103432597997,66.5244670539494,-21.8024606531298));
#24856=CARTESIAN_POINT('Ctrl Pts',(2.69285272661507,65.9264475450032,-23.5490026297785));
#24857=CARTESIAN_POINT('Ctrl Pts',(2.42604000771721,65.5973478982984,-24.4523631079317));
#24858=CARTESIAN_POINT('Ctrl Pts',(2.07963484569203,64.8987933787199,-26.2502710623803));
#24859=CARTESIAN_POINT('Ctrl Pts',(2.,64.5293013793053,-27.1447959433577));
#24860=CARTESIAN_POINT('Ctrl Pts',(2.,63.3502542343366,-29.846332338228));
#24861=CARTESIAN_POINT('Ctrl Pts',(2.38368127295869,62.4029020453759,-31.7791199130009));
#24862=CARTESIAN_POINT('Ctrl Pts',(3.90370579200787,60.4779252834904,-35.3051723987867));
#24863=CARTESIAN_POINT('Ctrl Pts',(5.03827663924619,59.503053899969,-36.9007032860843));
#24864=CARTESIAN_POINT('Ctrl Pts',(7.54764440420928,57.9574883058695,-39.2770767611709));
#24865=CARTESIAN_POINT('Ctrl Pts',(9.04077336951332,57.2551849551873,-40.2808837812864));
#24866=CARTESIAN_POINT('Ctrl Pts',(11.54482569449,56.5177517111439,-41.3027868899282));
#24867=CARTESIAN_POINT('Ctrl Pts',(12.4232339913984,56.3233853470359,-41.5658925850891));
#24868=CARTESIAN_POINT('Ctrl Pts',(14.2079498821129,56.064391561522,-41.9145698091276));
#24869=CARTESIAN_POINT('Ctrl Pts',(15.1143193052168,56.,-42.));
#24870=CARTESIAN_POINT('Ctrl Pts',(16.8856806947832,56.,-42.));
#24871=CARTESIAN_POINT('Ctrl Pts',(17.7920501178871,56.064391561522,-41.9145698091276));
#24872=CARTESIAN_POINT('Ctrl Pts',(19.5767660086016,56.3233853470359,-41.5658925850891));
#24873=CARTESIAN_POINT('Ctrl Pts',(20.45517430551,56.5177517111439,-41.3027868899282));
#24874=CARTESIAN_POINT('Ctrl Pts',(22.9592266304867,57.2551849551873,-40.2808837812864));
#24875=CARTESIAN_POINT('Ctrl Pts',(24.4523555957907,57.9574883058695,-39.2770767611709));
#24876=CARTESIAN_POINT('Ctrl Pts',(26.9617233607538,59.503053899969,-36.9007032860843));
#24877=CARTESIAN_POINT('Ctrl Pts',(28.0962942079921,60.4779252834904,-35.3051723987867));
#24878=CARTESIAN_POINT('Ctrl Pts',(29.6163187270413,62.4029020453759,-31.7791199130009));
#24879=CARTESIAN_POINT('Ctrl Pts',(30.,63.3502542343366,-29.846332338228));
#24880=CARTESIAN_POINT('Ctrl Pts',(30.,64.5293013793053,-27.1447959433577));
#24881=CARTESIAN_POINT('Ctrl Pts',(29.920365154308,64.8987933787199,-26.2502710623803));
#24882=CARTESIAN_POINT('Ctrl Pts',(29.5739599922828,65.5973478982984,-24.4523631079317));
#24883=CARTESIAN_POINT('Ctrl Pts',(29.3071472733849,65.9264475450032,-23.5490026297785));
#24884=CARTESIAN_POINT('Ctrl Pts',(28.58896567402,66.5244670539494,-21.8024606531298));
#24885=CARTESIAN_POINT('Ctrl Pts',(28.1369144367917,66.7940167052205,-20.9578499606675));
#24886=CARTESIAN_POINT('Ctrl Pts',(27.0781460846673,67.2665458430878,-19.3877268629585));
#24887=CARTESIAN_POINT('Ctrl Pts',(26.4713471796517,67.4697026576732,-18.662322985451));
#24888=CARTESIAN_POINT('Ctrl Pts',(24.5914812959786,67.9622849181329,-16.8132432389867));
#24889=CARTESIAN_POINT('Ctrl Pts',(23.0345575614708,68.2077217953467,-15.7551700622329));
#24890=CARTESIAN_POINT('Ctrl Pts',(20.6913501377322,68.4198540566006,-14.7917039729986));
#24891=CARTESIAN_POINT('Ctrl Pts',(20.038348684242,68.4654352022338,-14.5778037237174));
#24892=CARTESIAN_POINT('Ctrl Pts',(19.3775697035565,68.5,-14.4135353053998));
#24893=CARTESIAN_POINT('Origin',(16.,50.,-28.));
#24894=CARTESIAN_POINT('Origin',(16.,70.,-28.));
#24895=CARTESIAN_POINT('',(7.4,58.,-28.));
#24896=CARTESIAN_POINT('',(7.4,70.,-28.));
#24897=CARTESIAN_POINT('Origin',(16.,58.,-28.));
#24898=CARTESIAN_POINT('Origin',(16.,58.,-28.));
#24899=CARTESIAN_POINT('Origin',(0.4,-31.,-53.6935750346352));
#24900=CARTESIAN_POINT('',(35.5,-31.,-49.1935750346352));
#24901=CARTESIAN_POINT('',(0.4,-31.,-49.1935750346352));
#24902=CARTESIAN_POINT('Origin',(35.5,-31.,-53.6935750346352));
#24903=CARTESIAN_POINT('Origin',(0.4,62.,0.));
#24904=CARTESIAN_POINT('',(35.5,62.,4.5));
#24905=CARTESIAN_POINT('',(0.4,62.,4.5));
#24906=CARTESIAN_POINT('Origin',(35.5,62.,0.));
#24907=CARTESIAN_POINT('Origin',(0.4,31.,53.6935750346352));
#24908=CARTESIAN_POINT('',(35.5,31.,58.1935750346352));
#24909=CARTESIAN_POINT('',(0.4,31.,58.1935750346352));
#24910=CARTESIAN_POINT('Origin',(35.5,31.,53.6935750346352));
#24911=CARTESIAN_POINT('Origin',(0.4,-31.,53.6935750346352));
#24912=CARTESIAN_POINT('',(35.5,-31.,58.1935750346352));
#24913=CARTESIAN_POINT('',(0.4,-31.,58.1935750346352));
#24914=CARTESIAN_POINT('Origin',(35.5,-31.,53.6935750346352));
#24915=CARTESIAN_POINT('Origin',(0.4,-62.,7.59281015471359E-15));
#24916=CARTESIAN_POINT('',(35.5,-62.,4.50000000000001));
#24917=CARTESIAN_POINT('',(0.4,-62.,4.50000000000001));
#24918=CARTESIAN_POINT('Origin',(35.5,-62.,7.59281015471359E-15));
#24919=CARTESIAN_POINT('Origin',(0.4,31.,-53.6935750346352));
#24920=CARTESIAN_POINT('',(35.5,31.,-49.1935750346352));
#24921=CARTESIAN_POINT('',(0.4,31.,-49.1935750346352));
#24922=CARTESIAN_POINT('Origin',(35.5,31.,-53.6935750346352));
#24923=CARTESIAN_POINT('Origin',(10.25,0.,0.));
#24924=CARTESIAN_POINT('',(20.,-8.05,-9.85840673313619E-16));
#24925=CARTESIAN_POINT('Origin',(20.,0.,0.));
#24926=CARTESIAN_POINT('',(10.25,-8.05,-9.85840673313619E-16));
#24927=CARTESIAN_POINT('Origin',(35.,0.,0.));
#24928=CARTESIAN_POINT('',(35.5,-69.,-8.45006291411674E-15));
#24929=CARTESIAN_POINT('Origin',(35.5,0.,0.));
#24930=CARTESIAN_POINT('',(35.,-69.5,-8.51129525407411E-15));
#24931=CARTESIAN_POINT('Origin',(35.5,50.,0.));
#24932=CARTESIAN_POINT('',(35.5,-50.,-6.12323399573677E-15));
#24933=CARTESIAN_POINT('Origin',(35.5,0.,0.));
#24934=CARTESIAN_POINT('Origin',(30.75,0.,0.));
#24935=CARTESIAN_POINT('',(26.,-45.,-5.51091059616309E-15));
#24936=CARTESIAN_POINT('',(30.75,-47.5,-5.81707229594993E-15));
#24937=CARTESIAN_POINT('Origin',(26.,0.,0.));
#24938=CARTESIAN_POINT('Origin',(23.,0.,0.));
#24939=CARTESIAN_POINT('',(20.,-35.,-4.28626379701574E-15));
#24940=CARTESIAN_POINT('',(23.,-40.,-4.89858719658941E-15));
#24941=CARTESIAN_POINT('Origin',(20.,0.,0.));
#24942=CARTESIAN_POINT('Origin',(20.,8.05,0.));
#56599=UNCERTAINTY_MEASURE_WITH_UNIT(LENGTH_MEASURE(0.01),#56640,
'DISTANCE_ACCURACY_VALUE',
'Maximum model space distance between geometric entities at asserted c
onnectivities');
#56617=UNCERTAINTY_MEASURE_WITH_UNIT(LENGTH_MEASURE(0.01),#56640,
'DISTANCE_ACCURACY_VALUE',
'Maximum model space distance between geometric entities at asserted c
onnectivities');
#56621=(
GEOMETRIC_REPRESENTATION_CONTEXT(3)
GLOBAL_UNCERTAINTY_ASSIGNED_CONTEXT((#56599))
GLOBAL_UNIT_ASSIGNED_CONTEXT((#56640,#56642,#56643))
REPRESENTATION_CONTEXT('','3D')
);
#56639=(
GEOMETRIC_REPRESENTATION_CONTEXT(3)
GLOBAL_UNCERTAINTY_ASSIGNED_CONTEXT((#56617))
GLOBAL_UNIT_ASSIGNED_CONTEXT((#56640,#56642,#56643))
REPRESENTATION_CONTEXT('','3D')
);
#56640=(
LENGTH_UNIT()
NAMED_UNIT(*)
SI_UNIT(.MILLI.,.METRE.)
);
#56642=(
NAMED_UNIT(*)
PLANE_ANGLE_UNIT()
SI_UNIT($,.RADIAN.)
);
#56643=(
NAMED_UNIT(*)
SI_UNIT($,.STERADIAN.)
SOLID_ANGLE_UNIT()
);
#56647=SHAPE_DEFINITION_REPRESENTATION(#56668,#56747);
#56668=PRODUCT_DEFINITION_SHAPE('',$,#56769);
#56747=SHAPE_REPRESENTATION('',(#17536),#56621);
#56765=PRODUCT_DEFINITION_CONTEXT('part definition',#56830,'design');
#56769=PRODUCT_DEFINITION('2026-10-26-00-02-39-940',
'03_Center_Body_B_Exhaust',#56790,#56765);
#56790=PRODUCT_DEFINITION_FORMATION('',$,#56835);
#56830=APPLICATION_CONTEXT(
'Core Data for Automotive Mechanical Design Process');
#56831=PRODUCT_CONTEXT('part definition',#56830,'mechanical');
#56835=PRODUCT('2026-10-26-00-02-39-940','03_Center_Body_B_Exhaust',$,(#56831));
#56888=COLOUR_RGB('Dark Blue',0.08,0.2,0.34);
#56889=FILL_AREA_STYLE_COLOUR('',#56888);
#56890=FILL_AREA_STYLE('',(#56889));
#56891=SURFACE_STYLE_FILL_AREA(#56890);
#56892=SURFACE_SIDE_STYLE('',(#56891));
#56893=SURFACE_STYLE_USAGE(.BOTH.,#56892);
#56894=PRESENTATION_STYLE_ASSIGNMENT((#56893));
ENDSEC;
END-ISO-10303-21;
